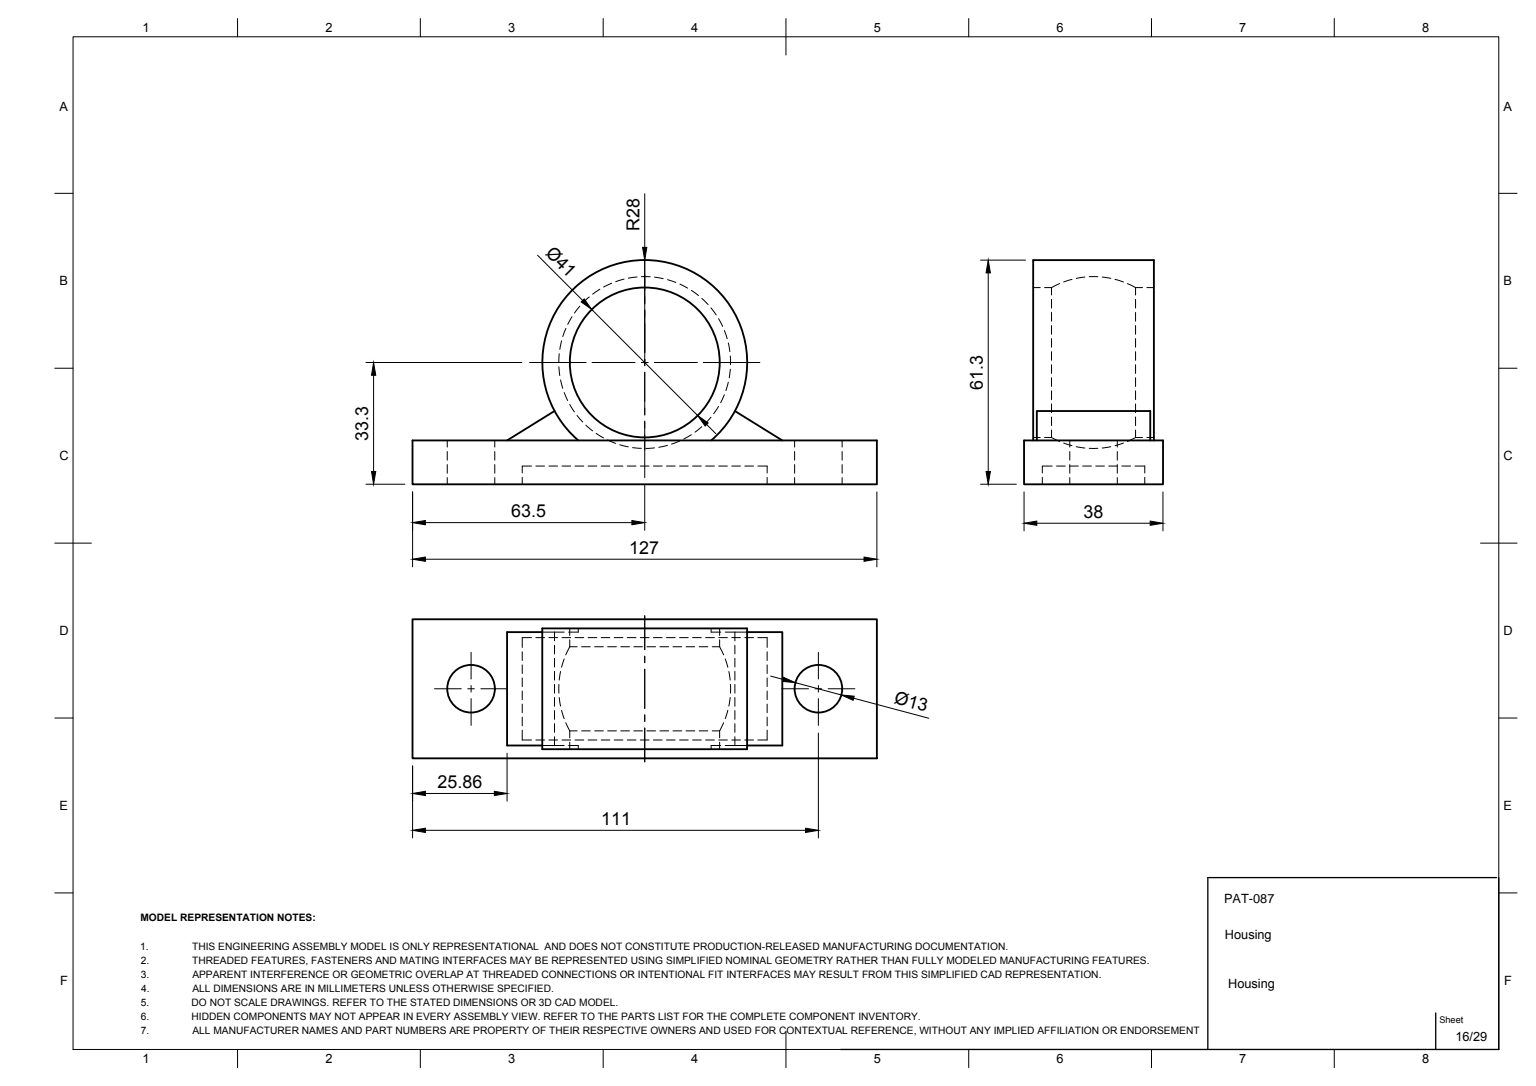
ISO-10303-21;
HEADER;
/* Generated by software containing ST-Developer
 * from STEP Tools, Inc. (www.steptools.com) 
 */

FILE_DESCRIPTION(
/* description */ ('Rigid flange shaft coupling assembly'),
/* implementation_level */ '2;1');

FILE_NAME(
/* name */ 'Housing.step',
/* time_stamp */ '2026-10-27T10:47:16-07:00',
/* author */ (''),
/* organization */ (''),
/* preprocessor_version */ 'ST-DEVELOPER v20.2',
/* originating_system */ 'Autodesk Translation Framework v15.17.0.0',
/* authorisation */ '');

FILE_SCHEMA (('AUTOMOTIVE_DESIGN { 1 0 10303 214 3 1 1 }'));
ENDSEC;

DATA;
#10=MECHANICAL_DESIGN_GEOMETRIC_PRESENTATION_REPRESENTATION('',(#407),#9141);
#340=SPHERICAL_SURFACE('',#5210,2.35);
#351=SHAPE_REPRESENTATION_RELATIONSHIP('SRR','None',#9286,#379);
#379=ADVANCED_BREP_SHAPE_REPRESENTATION('',(#436),#9121);
#407=STYLED_ITEM('',(#9479),#436);
#436=MANIFOLD_SOLID_BREP('Body1',#4761);
#485=FACE_BOUND('',#1109,.T.);
#486=FACE_BOUND('',#1110,.T.);
#487=FACE_BOUND('',#1118,.T.);
#488=FACE_BOUND('',#1119,.T.);
#489=FACE_BOUND('',#1120,.T.);
#490=FACE_BOUND('',#1123,.T.);
#491=FACE_BOUND('',#1125,.T.);
#492=FACE_BOUND('',#1138,.T.);
#493=FACE_BOUND('',#1139,.T.);
#494=FACE_BOUND('',#1140,.T.);
#608=PLANE('',#5212);
#609=PLANE('',#5214);
#610=PLANE('',#5216);
#611=PLANE('',#5218);
#612=PLANE('',#5219);
#613=PLANE('',#5221);
#614=PLANE('',#5222);
#615=PLANE('',#5228);
#616=PLANE('',#5229);
#617=PLANE('',#5230);
#618=PLANE('',#5231);
#619=PLANE('',#5232);
#620=PLANE('',#5233);
#621=PLANE('',#5234);
#622=PLANE('',#5239);
#623=PLANE('',#5240);
#624=PLANE('',#5241);
#625=PLANE('',#5242);
#626=PLANE('',#5243);
#802=FACE_OUTER_BOUND('',#1106,.T.);
#803=FACE_OUTER_BOUND('',#1107,.T.);
#804=FACE_OUTER_BOUND('',#1108,.T.);
#805=FACE_OUTER_BOUND('',#1111,.T.);
#806=FACE_OUTER_BOUND('',#1112,.T.);
#807=FACE_OUTER_BOUND('',#1113,.T.);
#808=FACE_OUTER_BOUND('',#1114,.T.);
#809=FACE_OUTER_BOUND('',#1115,.T.);
#810=FACE_OUTER_BOUND('',#1116,.T.);
#811=FACE_OUTER_BOUND('',#1117,.T.);
#812=FACE_OUTER_BOUND('',#1121,.T.);
#813=FACE_OUTER_BOUND('',#1122,.T.);
#814=FACE_OUTER_BOUND('',#1124,.T.);
#815=FACE_OUTER_BOUND('',#1126,.T.);
#816=FACE_OUTER_BOUND('',#1127,.T.);
#817=FACE_OUTER_BOUND('',#1128,.T.);
#818=FACE_OUTER_BOUND('',#1129,.T.);
#819=FACE_OUTER_BOUND('',#1130,.T.);
#820=FACE_OUTER_BOUND('',#1131,.T.);
#821=FACE_OUTER_BOUND('',#1132,.T.);
#822=FACE_OUTER_BOUND('',#1133,.T.);
#823=FACE_OUTER_BOUND('',#1134,.T.);
#824=FACE_OUTER_BOUND('',#1135,.T.);
#825=FACE_OUTER_BOUND('',#1136,.T.);
#826=FACE_OUTER_BOUND('',#1137,.T.);
#1106=EDGE_LOOP('',(#3483,#3484,#3485,#3486));
#1107=EDGE_LOOP('',(#3487,#3488,#3489,#3490));
#1108=EDGE_LOOP('',(#3491,#3492));
#1109=EDGE_LOOP('',(#3493));
#1110=EDGE_LOOP('',(#3494));
#1111=EDGE_LOOP('',(#3495,#3496,#3497));
#1112=EDGE_LOOP('',(#3498,#3499,#3500));
#1113=EDGE_LOOP('',(#3501,#3502,#3503));
#1114=EDGE_LOOP('',(#3504,#3505,#3506,#3507));
#1115=EDGE_LOOP('',(#3508,#3509,#3510));
#1116=EDGE_LOOP('',(#3511,#3512,#3513,#3514));
#1117=EDGE_LOOP('',(#3515,#3516,#3517,#3518));
#1118=EDGE_LOOP('',(#3519));
#1119=EDGE_LOOP('',(#3520));
#1120=EDGE_LOOP('',(#3521,#3522,#3523,#3524,#3525,#3526,#3527,#3528,#3529,
#3530,#3531,#3532));
#1121=EDGE_LOOP('',(#3533,#3534,#3535,#3536,#3537,#3538,#3539,#3540,#3541,
#3542,#3543,#3544));
#1122=EDGE_LOOP('',(#3545,#3546));
#1123=EDGE_LOOP('',(#3547));
#1124=EDGE_LOOP('',(#3548,#3549));
#1125=EDGE_LOOP('',(#3550));
#1126=EDGE_LOOP('',(#3551,#3552,#3553,#3554));
#1127=EDGE_LOOP('',(#3555,#3556,#3557,#3558));
#1128=EDGE_LOOP('',(#3559,#3560,#3561,#3562));
#1129=EDGE_LOOP('',(#3563,#3564,#3565,#3566));
#1130=EDGE_LOOP('',(#3567,#3568,#3569,#3570));
#1131=EDGE_LOOP('',(#3571,#3572,#3573,#3574));
#1132=EDGE_LOOP('',(#3575,#3576,#3577,#3578));
#1133=EDGE_LOOP('',(#3579,#3580,#3581,#3582));
#1134=EDGE_LOOP('',(#3583,#3584,#3585,#3586));
#1135=EDGE_LOOP('',(#3587,#3588,#3589,#3590));
#1136=EDGE_LOOP('',(#3591,#3592,#3593,#3594));
#1137=EDGE_LOOP('',(#3595,#3596,#3597,#3598));
#1138=EDGE_LOOP('',(#3599,#3600,#3601,#3602));
#1139=EDGE_LOOP('',(#3603));
#1140=EDGE_LOOP('',(#3604));
#1485=LINE('',#7360,#1830);
#1486=LINE('',#7366,#1831);
#1487=LINE('',#7375,#1832);
#1488=LINE('',#7377,#1833);
#1489=LINE('',#7382,#1834);
#1490=LINE('',#7385,#1835);
#1491=LINE('',#7389,#1836);
#1492=LINE('',#7392,#1837);
#1493=LINE('',#7394,#1838);
#1494=LINE('',#7395,#1839);
#1495=LINE('',#7399,#1840);
#1496=LINE('',#7401,#1841);
#1497=LINE('',#7404,#1842);
#1498=LINE('',#7405,#1843);
#1499=LINE('',#7409,#1844);
#1500=LINE('',#7411,#1845);
#1501=LINE('',#7413,#1846);
#1502=LINE('',#7414,#1847);
#1503=LINE('',#7420,#1848);
#1504=LINE('',#7422,#1849);
#1505=LINE('',#7423,#1850);
#1506=LINE('',#7425,#1851);
#1507=LINE('',#7427,#1852);
#1508=LINE('',#7428,#1853);
#1509=LINE('',#7437,#1854);
#1510=LINE('',#7439,#1855);
#1511=LINE('',#7441,#1856);
#1512=LINE('',#7442,#1857);
#1513=LINE('',#7445,#1858);
#1514=LINE('',#7447,#1859);
#1515=LINE('',#7448,#1860);
#1516=LINE('',#7451,#1861);
#1517=LINE('',#7453,#1862);
#1518=LINE('',#7454,#1863);
#1519=LINE('',#7456,#1864);
#1520=LINE('',#7457,#1865);
#1521=LINE('',#7462,#1866);
#1522=LINE('',#7466,#1867);
#1523=LINE('',#7470,#1868);
#1524=LINE('',#7471,#1869);
#1525=LINE('',#7472,#1870);
#1526=LINE('',#7475,#1871);
#1527=LINE('',#7476,#1872);
#1528=LINE('',#7479,#1873);
#1529=LINE('',#7480,#1874);
#1530=LINE('',#7482,#1875);
#1830=VECTOR('',#5948,2.05);
#1831=VECTOR('',#5955,2.05);
#1832=VECTOR('',#5964,1.);
#1833=VECTOR('',#5965,1.);
#1834=VECTOR('',#5970,1.);
#1835=VECTOR('',#5973,1.);
#1836=VECTOR('',#5976,1.);
#1837=VECTOR('',#5979,1.);
#1838=VECTOR('',#5982,1.);
#1839=VECTOR('',#5983,1.);
#1840=VECTOR('',#5986,1.);
#1841=VECTOR('',#5987,1.);
#1842=VECTOR('',#5992,1.);
#1843=VECTOR('',#5993,1.);
#1844=VECTOR('',#5996,1.);
#1845=VECTOR('',#5997,1.);
#1846=VECTOR('',#5998,1.);
#1847=VECTOR('',#5999,1.);
#1848=VECTOR('',#6004,1.);
#1849=VECTOR('',#6005,1.);
#1850=VECTOR('',#6006,1.);
#1851=VECTOR('',#6007,1.);
#1852=VECTOR('',#6008,1.);
#1853=VECTOR('',#6009,1.);
#1854=VECTOR('',#6022,1.);
#1855=VECTOR('',#6023,1.);
#1856=VECTOR('',#6024,1.);
#1857=VECTOR('',#6025,1.);
#1858=VECTOR('',#6028,1.);
#1859=VECTOR('',#6029,1.);
#1860=VECTOR('',#6030,1.);
#1861=VECTOR('',#6033,1.);
#1862=VECTOR('',#6034,1.);
#1863=VECTOR('',#6035,1.);
#1864=VECTOR('',#6038,1.);
#1865=VECTOR('',#6039,1.);
#1866=VECTOR('',#6046,0.65);
#1867=VECTOR('',#6051,0.65);
#1868=VECTOR('',#6054,1.);
#1869=VECTOR('',#6055,1.);
#1870=VECTOR('',#6056,1.);
#1871=VECTOR('',#6059,1.);
#1872=VECTOR('',#6060,1.);
#1873=VECTOR('',#6063,1.);
#1874=VECTOR('',#6064,1.);
#1875=VECTOR('',#6067,1.);
#2135=CIRCLE('',#5205,2.05);
#2136=CIRCLE('',#5206,2.05);
#2137=CIRCLE('',#5208,2.05);
#2138=CIRCLE('',#5209,2.05);
#2139=CIRCLE('',#5211,2.35);
#2140=CIRCLE('',#5213,2.8);
#2141=CIRCLE('',#5215,2.8);
#2142=CIRCLE('',#5217,2.8);
#2143=CIRCLE('',#5220,2.8);
#2144=CIRCLE('',#5223,0.65);
#2145=CIRCLE('',#5224,0.65);
#2146=CIRCLE('',#5226,2.8);
#2147=CIRCLE('',#5227,2.8);
#2148=CIRCLE('',#5236,0.65);
#2149=CIRCLE('',#5238,0.65);
#2356=VERTEX_POINT('',#7357);
#2357=VERTEX_POINT('',#7359);
#2358=VERTEX_POINT('',#7363);
#2359=VERTEX_POINT('',#7365);
#2360=VERTEX_POINT('',#7369);
#2361=VERTEX_POINT('',#7370);
#2362=VERTEX_POINT('',#7373);
#2363=VERTEX_POINT('',#7374);
#2364=VERTEX_POINT('',#7376);
#2365=VERTEX_POINT('',#7380);
#2366=VERTEX_POINT('',#7381);
#2367=VERTEX_POINT('',#7383);
#2368=VERTEX_POINT('',#7387);
#2369=VERTEX_POINT('',#7388);
#2370=VERTEX_POINT('',#7390);
#2371=VERTEX_POINT('',#7397);
#2372=VERTEX_POINT('',#7398);
#2373=VERTEX_POINT('',#7400);
#2374=VERTEX_POINT('',#7407);
#2375=VERTEX_POINT('',#7408);
#2376=VERTEX_POINT('',#7410);
#2377=VERTEX_POINT('',#7412);
#2378=VERTEX_POINT('',#7415);
#2379=VERTEX_POINT('',#7417);
#2380=VERTEX_POINT('',#7419);
#2381=VERTEX_POINT('',#7421);
#2382=VERTEX_POINT('',#7424);
#2383=VERTEX_POINT('',#7426);
#2384=VERTEX_POINT('',#7435);
#2385=VERTEX_POINT('',#7436);
#2386=VERTEX_POINT('',#7438);
#2387=VERTEX_POINT('',#7440);
#2388=VERTEX_POINT('',#7444);
#2389=VERTEX_POINT('',#7446);
#2390=VERTEX_POINT('',#7450);
#2391=VERTEX_POINT('',#7452);
#2392=VERTEX_POINT('',#7460);
#2393=VERTEX_POINT('',#7464);
#2394=VERTEX_POINT('',#7468);
#2395=VERTEX_POINT('',#7469);
#2396=VERTEX_POINT('',#7474);
#2397=VERTEX_POINT('',#7478);
#2785=EDGE_CURVE('',#2356,#2356,#2135,.T.);
#2786=EDGE_CURVE('',#2356,#2357,#1485,.T.);
#2787=EDGE_CURVE('',#2357,#2357,#2136,.T.);
#2788=EDGE_CURVE('',#2358,#2358,#2137,.T.);
#2789=EDGE_CURVE('',#2358,#2359,#1486,.T.);
#2790=EDGE_CURVE('',#2359,#2359,#2138,.T.);
#2791=EDGE_CURVE('',#2360,#2361,#2139,.T.);
#2792=EDGE_CURVE('',#2362,#2363,#1487,.T.);
#2793=EDGE_CURVE('',#2362,#2364,#1488,.T.);
#2794=EDGE_CURVE('',#2363,#2364,#2140,.T.);
#2795=EDGE_CURVE('',#2365,#2366,#1489,.T.);
#2796=EDGE_CURVE('',#2367,#2365,#2141,.T.);
#2797=EDGE_CURVE('',#2367,#2366,#1490,.T.);
#2798=EDGE_CURVE('',#2368,#2369,#1491,.T.);
#2799=EDGE_CURVE('',#2370,#2368,#2142,.T.);
#2800=EDGE_CURVE('',#2370,#2369,#1492,.T.);
#2801=EDGE_CURVE('',#2369,#2362,#1493,.T.);
#2802=EDGE_CURVE('',#2364,#2370,#1494,.T.);
#2803=EDGE_CURVE('',#2371,#2372,#1495,.T.);
#2804=EDGE_CURVE('',#2371,#2373,#1496,.T.);
#2805=EDGE_CURVE('',#2372,#2373,#2143,.T.);
#2806=EDGE_CURVE('',#2366,#2371,#1497,.T.);
#2807=EDGE_CURVE('',#2373,#2367,#1498,.T.);
#2808=EDGE_CURVE('',#2374,#2375,#1499,.T.);
#2809=EDGE_CURVE('',#2375,#2376,#1500,.T.);
#2810=EDGE_CURVE('',#2376,#2377,#1501,.T.);
#2811=EDGE_CURVE('',#2377,#2374,#1502,.T.);
#2812=EDGE_CURVE('',#2378,#2378,#2144,.T.);
#2813=EDGE_CURVE('',#2379,#2379,#2145,.T.);
#2814=EDGE_CURVE('',#2372,#2380,#1503,.T.);
#2815=EDGE_CURVE('',#2380,#2381,#1504,.T.);
#2816=EDGE_CURVE('',#2381,#2368,#1505,.T.);
#2817=EDGE_CURVE('',#2363,#2382,#1506,.T.);
#2818=EDGE_CURVE('',#2382,#2383,#1507,.T.);
#2819=EDGE_CURVE('',#2383,#2365,#1508,.T.);
#2820=EDGE_CURVE('',#2382,#2383,#2146,.T.);
#2821=EDGE_CURVE('',#2380,#2381,#2147,.T.);
#2822=EDGE_CURVE('',#2384,#2385,#1509,.T.);
#2823=EDGE_CURVE('',#2384,#2386,#1510,.T.);
#2824=EDGE_CURVE('',#2386,#2387,#1511,.T.);
#2825=EDGE_CURVE('',#2385,#2387,#1512,.T.);
#2826=EDGE_CURVE('',#2388,#2384,#1513,.T.);
#2827=EDGE_CURVE('',#2388,#2389,#1514,.T.);
#2828=EDGE_CURVE('',#2389,#2386,#1515,.T.);
#2829=EDGE_CURVE('',#2390,#2388,#1516,.T.);
#2830=EDGE_CURVE('',#2390,#2391,#1517,.T.);
#2831=EDGE_CURVE('',#2391,#2389,#1518,.T.);
#2832=EDGE_CURVE('',#2385,#2390,#1519,.T.);
#2833=EDGE_CURVE('',#2387,#2391,#1520,.T.);
#2834=EDGE_CURVE('',#2392,#2392,#2148,.T.);
#2835=EDGE_CURVE('',#2392,#2379,#1521,.T.);
#2836=EDGE_CURVE('',#2393,#2393,#2149,.T.);
#2837=EDGE_CURVE('',#2393,#2378,#1522,.T.);
#2838=EDGE_CURVE('',#2394,#2395,#1523,.T.);
#2839=EDGE_CURVE('',#2395,#2374,#1524,.T.);
#2840=EDGE_CURVE('',#2394,#2377,#1525,.T.);
#2841=EDGE_CURVE('',#2396,#2394,#1526,.T.);
#2842=EDGE_CURVE('',#2396,#2376,#1527,.T.);
#2843=EDGE_CURVE('',#2397,#2396,#1528,.T.);
#2844=EDGE_CURVE('',#2397,#2375,#1529,.T.);
#2845=EDGE_CURVE('',#2395,#2397,#1530,.T.);
#3483=ORIENTED_EDGE('',*,*,#2785,.F.);
#3484=ORIENTED_EDGE('',*,*,#2786,.T.);
#3485=ORIENTED_EDGE('',*,*,#2787,.F.);
#3486=ORIENTED_EDGE('',*,*,#2786,.F.);
#3487=ORIENTED_EDGE('',*,*,#2788,.F.);
#3488=ORIENTED_EDGE('',*,*,#2789,.T.);
#3489=ORIENTED_EDGE('',*,*,#2790,.F.);
#3490=ORIENTED_EDGE('',*,*,#2789,.F.);
#3491=ORIENTED_EDGE('',*,*,#2791,.T.);
#3492=ORIENTED_EDGE('',*,*,#2791,.F.);
#3493=ORIENTED_EDGE('',*,*,#2788,.T.);
#3494=ORIENTED_EDGE('',*,*,#2787,.T.);
#3495=ORIENTED_EDGE('',*,*,#2792,.F.);
#3496=ORIENTED_EDGE('',*,*,#2793,.T.);
#3497=ORIENTED_EDGE('',*,*,#2794,.F.);
#3498=ORIENTED_EDGE('',*,*,#2795,.F.);
#3499=ORIENTED_EDGE('',*,*,#2796,.F.);
#3500=ORIENTED_EDGE('',*,*,#2797,.T.);
#3501=ORIENTED_EDGE('',*,*,#2798,.F.);
#3502=ORIENTED_EDGE('',*,*,#2799,.F.);
#3503=ORIENTED_EDGE('',*,*,#2800,.T.);
#3504=ORIENTED_EDGE('',*,*,#2801,.F.);
#3505=ORIENTED_EDGE('',*,*,#2800,.F.);
#3506=ORIENTED_EDGE('',*,*,#2802,.F.);
#3507=ORIENTED_EDGE('',*,*,#2793,.F.);
#3508=ORIENTED_EDGE('',*,*,#2803,.F.);
#3509=ORIENTED_EDGE('',*,*,#2804,.T.);
#3510=ORIENTED_EDGE('',*,*,#2805,.F.);
#3511=ORIENTED_EDGE('',*,*,#2806,.F.);
#3512=ORIENTED_EDGE('',*,*,#2797,.F.);
#3513=ORIENTED_EDGE('',*,*,#2807,.F.);
#3514=ORIENTED_EDGE('',*,*,#2804,.F.);
#3515=ORIENTED_EDGE('',*,*,#2808,.T.);
#3516=ORIENTED_EDGE('',*,*,#2809,.T.);
#3517=ORIENTED_EDGE('',*,*,#2810,.T.);
#3518=ORIENTED_EDGE('',*,*,#2811,.T.);
#3519=ORIENTED_EDGE('',*,*,#2812,.T.);
#3520=ORIENTED_EDGE('',*,*,#2813,.T.);
#3521=ORIENTED_EDGE('',*,*,#2795,.T.);
#3522=ORIENTED_EDGE('',*,*,#2806,.T.);
#3523=ORIENTED_EDGE('',*,*,#2803,.T.);
#3524=ORIENTED_EDGE('',*,*,#2814,.T.);
#3525=ORIENTED_EDGE('',*,*,#2815,.T.);
#3526=ORIENTED_EDGE('',*,*,#2816,.T.);
#3527=ORIENTED_EDGE('',*,*,#2798,.T.);
#3528=ORIENTED_EDGE('',*,*,#2801,.T.);
#3529=ORIENTED_EDGE('',*,*,#2792,.T.);
#3530=ORIENTED_EDGE('',*,*,#2817,.T.);
#3531=ORIENTED_EDGE('',*,*,#2818,.T.);
#3532=ORIENTED_EDGE('',*,*,#2819,.T.);
#3533=ORIENTED_EDGE('',*,*,#2796,.T.);
#3534=ORIENTED_EDGE('',*,*,#2819,.F.);
#3535=ORIENTED_EDGE('',*,*,#2820,.F.);
#3536=ORIENTED_EDGE('',*,*,#2817,.F.);
#3537=ORIENTED_EDGE('',*,*,#2794,.T.);
#3538=ORIENTED_EDGE('',*,*,#2802,.T.);
#3539=ORIENTED_EDGE('',*,*,#2799,.T.);
#3540=ORIENTED_EDGE('',*,*,#2816,.F.);
#3541=ORIENTED_EDGE('',*,*,#2821,.F.);
#3542=ORIENTED_EDGE('',*,*,#2814,.F.);
#3543=ORIENTED_EDGE('',*,*,#2805,.T.);
#3544=ORIENTED_EDGE('',*,*,#2807,.T.);
#3545=ORIENTED_EDGE('',*,*,#2815,.F.);
#3546=ORIENTED_EDGE('',*,*,#2821,.T.);
#3547=ORIENTED_EDGE('',*,*,#2785,.T.);
#3548=ORIENTED_EDGE('',*,*,#2818,.F.);
#3549=ORIENTED_EDGE('',*,*,#2820,.T.);
#3550=ORIENTED_EDGE('',*,*,#2790,.T.);
#3551=ORIENTED_EDGE('',*,*,#2822,.F.);
#3552=ORIENTED_EDGE('',*,*,#2823,.T.);
#3553=ORIENTED_EDGE('',*,*,#2824,.T.);
#3554=ORIENTED_EDGE('',*,*,#2825,.F.);
#3555=ORIENTED_EDGE('',*,*,#2826,.F.);
#3556=ORIENTED_EDGE('',*,*,#2827,.T.);
#3557=ORIENTED_EDGE('',*,*,#2828,.T.);
#3558=ORIENTED_EDGE('',*,*,#2823,.F.);
#3559=ORIENTED_EDGE('',*,*,#2829,.F.);
#3560=ORIENTED_EDGE('',*,*,#2830,.T.);
#3561=ORIENTED_EDGE('',*,*,#2831,.T.);
#3562=ORIENTED_EDGE('',*,*,#2827,.F.);
#3563=ORIENTED_EDGE('',*,*,#2832,.F.);
#3564=ORIENTED_EDGE('',*,*,#2825,.T.);
#3565=ORIENTED_EDGE('',*,*,#2833,.T.);
#3566=ORIENTED_EDGE('',*,*,#2830,.F.);
#3567=ORIENTED_EDGE('',*,*,#2833,.F.);
#3568=ORIENTED_EDGE('',*,*,#2824,.F.);
#3569=ORIENTED_EDGE('',*,*,#2828,.F.);
#3570=ORIENTED_EDGE('',*,*,#2831,.F.);
#3571=ORIENTED_EDGE('',*,*,#2834,.F.);
#3572=ORIENTED_EDGE('',*,*,#2835,.T.);
#3573=ORIENTED_EDGE('',*,*,#2813,.F.);
#3574=ORIENTED_EDGE('',*,*,#2835,.F.);
#3575=ORIENTED_EDGE('',*,*,#2836,.F.);
#3576=ORIENTED_EDGE('',*,*,#2837,.T.);
#3577=ORIENTED_EDGE('',*,*,#2812,.F.);
#3578=ORIENTED_EDGE('',*,*,#2837,.F.);
#3579=ORIENTED_EDGE('',*,*,#2838,.T.);
#3580=ORIENTED_EDGE('',*,*,#2839,.T.);
#3581=ORIENTED_EDGE('',*,*,#2811,.F.);
#3582=ORIENTED_EDGE('',*,*,#2840,.F.);
#3583=ORIENTED_EDGE('',*,*,#2841,.T.);
#3584=ORIENTED_EDGE('',*,*,#2840,.T.);
#3585=ORIENTED_EDGE('',*,*,#2810,.F.);
#3586=ORIENTED_EDGE('',*,*,#2842,.F.);
#3587=ORIENTED_EDGE('',*,*,#2843,.T.);
#3588=ORIENTED_EDGE('',*,*,#2842,.T.);
#3589=ORIENTED_EDGE('',*,*,#2809,.F.);
#3590=ORIENTED_EDGE('',*,*,#2844,.F.);
#3591=ORIENTED_EDGE('',*,*,#2845,.T.);
#3592=ORIENTED_EDGE('',*,*,#2844,.T.);
#3593=ORIENTED_EDGE('',*,*,#2808,.F.);
#3594=ORIENTED_EDGE('',*,*,#2839,.F.);
#3595=ORIENTED_EDGE('',*,*,#2845,.F.);
#3596=ORIENTED_EDGE('',*,*,#2838,.F.);
#3597=ORIENTED_EDGE('',*,*,#2841,.F.);
#3598=ORIENTED_EDGE('',*,*,#2843,.F.);
#3599=ORIENTED_EDGE('',*,*,#2822,.T.);
#3600=ORIENTED_EDGE('',*,*,#2832,.T.);
#3601=ORIENTED_EDGE('',*,*,#2829,.T.);
#3602=ORIENTED_EDGE('',*,*,#2826,.T.);
#3603=ORIENTED_EDGE('',*,*,#2834,.T.);
#3604=ORIENTED_EDGE('',*,*,#2836,.T.);
#4419=CYLINDRICAL_SURFACE('',#5204,2.05);
#4420=CYLINDRICAL_SURFACE('',#5207,2.05);
#4421=CYLINDRICAL_SURFACE('',#5225,2.8);
#4422=CYLINDRICAL_SURFACE('',#5235,0.65);
#4423=CYLINDRICAL_SURFACE('',#5237,0.65);
#4538=ADVANCED_FACE('',(#802),#4419,.F.);
#4539=ADVANCED_FACE('',(#803),#4420,.F.);
#4540=ADVANCED_FACE('',(#804,#485,#486),#340,.F.);
#4541=ADVANCED_FACE('',(#805),#608,.T.);
#4542=ADVANCED_FACE('',(#806),#609,.T.);
#4543=ADVANCED_FACE('',(#807),#610,.T.);
#4544=ADVANCED_FACE('',(#808),#611,.T.);
#4545=ADVANCED_FACE('',(#809),#612,.T.);
#4546=ADVANCED_FACE('',(#810),#613,.T.);
#4547=ADVANCED_FACE('',(#811,#487,#488,#489),#614,.T.);
#4548=ADVANCED_FACE('',(#812),#4421,.T.);
#4549=ADVANCED_FACE('',(#813,#490),#615,.F.);
#4550=ADVANCED_FACE('',(#814,#491),#616,.T.);
#4551=ADVANCED_FACE('',(#815),#617,.F.);
#4552=ADVANCED_FACE('',(#816),#618,.F.);
#4553=ADVANCED_FACE('',(#817),#619,.F.);
#4554=ADVANCED_FACE('',(#818),#620,.F.);
#4555=ADVANCED_FACE('',(#819),#621,.F.);
#4556=ADVANCED_FACE('',(#820),#4422,.F.);
#4557=ADVANCED_FACE('',(#821),#4423,.F.);
#4558=ADVANCED_FACE('',(#822),#622,.T.);
#4559=ADVANCED_FACE('',(#823),#623,.T.);
#4560=ADVANCED_FACE('',(#824),#624,.T.);
#4561=ADVANCED_FACE('',(#825),#625,.T.);
#4562=ADVANCED_FACE('',(#826,#492,#493,#494),#626,.F.);
#4761=CLOSED_SHELL('',(#4538,#4539,#4540,#4541,#4542,#4543,#4544,#4545,
#4546,#4547,#4548,#4549,#4550,#4551,#4552,#4553,#4554,#4555,#4556,#4557,
#4558,#4559,#4560,#4561,#4562));
#5203=AXIS2_PLACEMENT_3D('',#7355,#5942,#5943);
#5204=AXIS2_PLACEMENT_3D('',#7356,#5944,#5945);
#5205=AXIS2_PLACEMENT_3D('',#7358,#5946,#5947);
#5206=AXIS2_PLACEMENT_3D('',#7361,#5949,#5950);
#5207=AXIS2_PLACEMENT_3D('',#7362,#5951,#5952);
#5208=AXIS2_PLACEMENT_3D('',#7364,#5953,#5954);
#5209=AXIS2_PLACEMENT_3D('',#7367,#5956,#5957);
#5210=AXIS2_PLACEMENT_3D('',#7368,#5958,#5959);
#5211=AXIS2_PLACEMENT_3D('',#7371,#5960,#5961);
#5212=AXIS2_PLACEMENT_3D('',#7372,#5962,#5963);
#5213=AXIS2_PLACEMENT_3D('',#7378,#5966,#5967);
#5214=AXIS2_PLACEMENT_3D('',#7379,#5968,#5969);
#5215=AXIS2_PLACEMENT_3D('',#7384,#5971,#5972);
#5216=AXIS2_PLACEMENT_3D('',#7386,#5974,#5975);
#5217=AXIS2_PLACEMENT_3D('',#7391,#5977,#5978);
#5218=AXIS2_PLACEMENT_3D('',#7393,#5980,#5981);
#5219=AXIS2_PLACEMENT_3D('',#7396,#5984,#5985);
#5220=AXIS2_PLACEMENT_3D('',#7402,#5988,#5989);
#5221=AXIS2_PLACEMENT_3D('',#7403,#5990,#5991);
#5222=AXIS2_PLACEMENT_3D('',#7406,#5994,#5995);
#5223=AXIS2_PLACEMENT_3D('',#7416,#6000,#6001);
#5224=AXIS2_PLACEMENT_3D('',#7418,#6002,#6003);
#5225=AXIS2_PLACEMENT_3D('',#7429,#6010,#6011);
#5226=AXIS2_PLACEMENT_3D('',#7430,#6012,#6013);
#5227=AXIS2_PLACEMENT_3D('',#7431,#6014,#6015);
#5228=AXIS2_PLACEMENT_3D('',#7432,#6016,#6017);
#5229=AXIS2_PLACEMENT_3D('',#7433,#6018,#6019);
#5230=AXIS2_PLACEMENT_3D('',#7434,#6020,#6021);
#5231=AXIS2_PLACEMENT_3D('',#7443,#6026,#6027);
#5232=AXIS2_PLACEMENT_3D('',#7449,#6031,#6032);
#5233=AXIS2_PLACEMENT_3D('',#7455,#6036,#6037);
#5234=AXIS2_PLACEMENT_3D('',#7458,#6040,#6041);
#5235=AXIS2_PLACEMENT_3D('',#7459,#6042,#6043);
#5236=AXIS2_PLACEMENT_3D('',#7461,#6044,#6045);
#5237=AXIS2_PLACEMENT_3D('',#7463,#6047,#6048);
#5238=AXIS2_PLACEMENT_3D('',#7465,#6049,#6050);
#5239=AXIS2_PLACEMENT_3D('',#7467,#6052,#6053);
#5240=AXIS2_PLACEMENT_3D('',#7473,#6057,#6058);
#5241=AXIS2_PLACEMENT_3D('',#7477,#6061,#6062);
#5242=AXIS2_PLACEMENT_3D('',#7481,#6065,#6066);
#5243=AXIS2_PLACEMENT_3D('',#7483,#6068,#6069);
#5942=DIRECTION('axis',(0.,0.,1.));
#5943=DIRECTION('refdir',(1.,0.,0.));
#5944=DIRECTION('center_axis',(0.,1.,0.));
#5945=DIRECTION('ref_axis',(1.,0.,0.));
#5946=DIRECTION('center_axis',(0.,1.,0.));
#5947=DIRECTION('ref_axis',(1.,0.,0.));
#5948=DIRECTION('',(0.,1.,0.));
#5949=DIRECTION('center_axis',(0.,-1.,0.));
#5950=DIRECTION('ref_axis',(1.,0.,0.));
#5951=DIRECTION('center_axis',(0.,1.,0.));
#5952=DIRECTION('ref_axis',(1.,0.,0.));
#5953=DIRECTION('center_axis',(0.,1.,0.));
#5954=DIRECTION('ref_axis',(1.,0.,0.));
#5955=DIRECTION('',(0.,1.,0.));
#5956=DIRECTION('center_axis',(0.,-1.,0.));
#5957=DIRECTION('ref_axis',(1.,0.,0.));
#5958=DIRECTION('center_axis',(6.12323399573677E-17,0.,1.));
#5959=DIRECTION('ref_axis',(1.,0.,0.));
#5960=DIRECTION('center_axis',(-1.22464679914735E-16,1.,0.));
#5961=DIRECTION('ref_axis',(-1.,-1.22464679914735E-16,0.));
#5962=DIRECTION('center_axis',(0.,1.,0.));
#5963=DIRECTION('ref_axis',(0.,0.,1.));
#5964=DIRECTION('',(1.,0.,0.));
#5965=DIRECTION('',(0.850265146687862,0.,0.526354614616295));
#5966=DIRECTION('center_axis',(0.,1.,0.));
#5967=DIRECTION('ref_axis',(1.,0.,0.));
#5968=DIRECTION('center_axis',(0.,1.,0.));
#5969=DIRECTION('ref_axis',(0.,0.,1.));
#5970=DIRECTION('',(1.,0.,0.));
#5971=DIRECTION('center_axis',(0.,1.,0.));
#5972=DIRECTION('ref_axis',(1.,0.,0.));
#5973=DIRECTION('',(0.850265146687862,0.,-0.526354614616295));
#5974=DIRECTION('center_axis',(0.,-1.,0.));
#5975=DIRECTION('ref_axis',(0.,0.,-1.));
#5976=DIRECTION('',(-1.,0.,0.));
#5977=DIRECTION('center_axis',(0.,-1.,0.));
#5978=DIRECTION('ref_axis',(1.,0.,0.));
#5979=DIRECTION('',(-0.850265146687862,0.,-0.526354614616295));
#5980=DIRECTION('center_axis',(-0.526354614616295,0.,0.850265146687862));
#5981=DIRECTION('ref_axis',(0.850265146687862,0.,0.526354614616295));
#5982=DIRECTION('',(0.,1.,0.));
#5983=DIRECTION('',(0.,-1.,0.));
#5984=DIRECTION('center_axis',(0.,-1.,0.));
#5985=DIRECTION('ref_axis',(0.,0.,-1.));
#5986=DIRECTION('',(-1.,0.,0.));
#5987=DIRECTION('',(-0.850265146687862,0.,0.526354614616295));
#5988=DIRECTION('center_axis',(0.,-1.,0.));
#5989=DIRECTION('ref_axis',(1.,0.,0.));
#5990=DIRECTION('center_axis',(0.526354614616295,0.,0.850265146687862));
#5991=DIRECTION('ref_axis',(0.850265146687862,0.,-0.526354614616295));
#5992=DIRECTION('',(0.,-1.,0.));
#5993=DIRECTION('',(0.,1.,0.));
#5994=DIRECTION('center_axis',(0.,0.,1.));
#5995=DIRECTION('ref_axis',(1.,0.,0.));
#5996=DIRECTION('',(0.,-1.,0.));
#5997=DIRECTION('',(1.,0.,0.));
#5998=DIRECTION('',(0.,1.,0.));
#5999=DIRECTION('',(-1.,0.,0.));
#6000=DIRECTION('center_axis',(0.,0.,-1.));
#6001=DIRECTION('ref_axis',(1.,0.,0.));
#6002=DIRECTION('center_axis',(0.,0.,-1.));
#6003=DIRECTION('ref_axis',(1.,0.,0.));
#6004=DIRECTION('',(0.,-1.,0.));
#6005=DIRECTION('',(-1.,0.,0.));
#6006=DIRECTION('',(0.,1.,0.));
#6007=DIRECTION('',(0.,1.,0.));
#6008=DIRECTION('',(1.,0.,0.));
#6009=DIRECTION('',(0.,-1.,0.));
#6010=DIRECTION('center_axis',(0.,1.,0.));
#6011=DIRECTION('ref_axis',(6.12323399573677E-17,0.,1.));
#6012=DIRECTION('center_axis',(0.,1.,0.));
#6013=DIRECTION('ref_axis',(1.,0.,0.));
#6014=DIRECTION('center_axis',(0.,-1.,0.));
#6015=DIRECTION('ref_axis',(1.,0.,0.));
#6016=DIRECTION('center_axis',(0.,1.,0.));
#6017=DIRECTION('ref_axis',(1.,0.,0.));
#6018=DIRECTION('center_axis',(0.,1.,0.));
#6019=DIRECTION('ref_axis',(1.,0.,0.));
#6020=DIRECTION('center_axis',(0.,1.,0.));
#6021=DIRECTION('ref_axis',(-1.,0.,0.));
#6022=DIRECTION('',(-1.,0.,0.));
#6023=DIRECTION('',(0.,0.,1.));
#6024=DIRECTION('',(-1.,0.,0.));
#6025=DIRECTION('',(0.,0.,1.));
#6026=DIRECTION('center_axis',(1.,0.,0.));
#6027=DIRECTION('ref_axis',(0.,1.,0.));
#6028=DIRECTION('',(0.,1.,0.));
#6029=DIRECTION('',(0.,0.,1.));
#6030=DIRECTION('',(0.,1.,0.));
#6031=DIRECTION('center_axis',(0.,-1.,0.));
#6032=DIRECTION('ref_axis',(1.,0.,0.));
#6033=DIRECTION('',(1.,0.,0.));
#6034=DIRECTION('',(0.,0.,1.));
#6035=DIRECTION('',(1.,0.,0.));
#6036=DIRECTION('center_axis',(-1.,0.,0.));
#6037=DIRECTION('ref_axis',(0.,-1.,0.));
#6038=DIRECTION('',(0.,-1.,0.));
#6039=DIRECTION('',(0.,-1.,0.));
#6040=DIRECTION('center_axis',(0.,0.,1.));
#6041=DIRECTION('ref_axis',(1.,0.,0.));
#6042=DIRECTION('center_axis',(0.,0.,1.));
#6043=DIRECTION('ref_axis',(1.,0.,0.));
#6044=DIRECTION('center_axis',(0.,0.,1.));
#6045=DIRECTION('ref_axis',(1.,0.,0.));
#6046=DIRECTION('',(0.,0.,1.));
#6047=DIRECTION('center_axis',(0.,0.,1.));
#6048=DIRECTION('ref_axis',(1.,0.,0.));
#6049=DIRECTION('center_axis',(0.,0.,1.));
#6050=DIRECTION('ref_axis',(1.,0.,0.));
#6051=DIRECTION('',(0.,0.,1.));
#6052=DIRECTION('center_axis',(0.,1.,0.));
#6053=DIRECTION('ref_axis',(-1.,0.,0.));
#6054=DIRECTION('',(-1.,0.,0.));
#6055=DIRECTION('',(0.,0.,1.));
#6056=DIRECTION('',(0.,0.,1.));
#6057=DIRECTION('center_axis',(1.,0.,0.));
#6058=DIRECTION('ref_axis',(0.,1.,0.));
#6059=DIRECTION('',(0.,1.,0.));
#6060=DIRECTION('',(0.,0.,1.));
#6061=DIRECTION('center_axis',(0.,-1.,0.));
#6062=DIRECTION('ref_axis',(1.,0.,0.));
#6063=DIRECTION('',(1.,0.,0.));
#6064=DIRECTION('',(0.,0.,1.));
#6065=DIRECTION('center_axis',(-1.,0.,0.));
#6066=DIRECTION('ref_axis',(0.,-1.,0.));
#6067=DIRECTION('',(0.,-1.,0.));
#6068=DIRECTION('center_axis',(0.,0.,1.));
#6069=DIRECTION('ref_axis',(1.,0.,0.));
#7355=CARTESIAN_POINT('',(0.,0.,0.));
#7356=CARTESIAN_POINT('Origin',(0.,0.,0.));
#7357=CARTESIAN_POINT('',(-2.05,-1.65,2.51052593825207E-16));
#7358=CARTESIAN_POINT('Origin',(0.,-1.65,0.));
#7359=CARTESIAN_POINT('',(-2.05,-1.14891252930761,-2.51052593825207E-16));
#7360=CARTESIAN_POINT('',(-2.05,0.,2.51052593825207E-16));
#7361=CARTESIAN_POINT('Origin',(0.,-1.14891252930761,0.));
#7362=CARTESIAN_POINT('Origin',(0.,0.,0.));
#7363=CARTESIAN_POINT('',(-2.05,1.14891252930761,2.51052593825207E-16));
#7364=CARTESIAN_POINT('Origin',(0.,1.14891252930761,0.));
#7365=CARTESIAN_POINT('',(-2.05,1.65,-2.51052593825207E-16));
#7366=CARTESIAN_POINT('',(-2.05,0.,2.51052593825207E-16));
#7367=CARTESIAN_POINT('Origin',(0.,1.65,0.));
#7368=CARTESIAN_POINT('Origin',(0.,0.,0.));
#7369=CARTESIAN_POINT('',(-1.43895998899814E-16,-1.76221774462768E-32,-2.35));
#7370=CARTESIAN_POINT('',(-1.43895998899814E-16,-1.76221774462768E-32,2.35));
#7371=CARTESIAN_POINT('Origin',(0.,0.,0.));
#7372=CARTESIAN_POINT('Origin',(0.,1.55,-1.49));
#7373=CARTESIAN_POINT('',(-3.76384615384615,1.55,-2.13));
#7374=CARTESIAN_POINT('',(-1.81744325908679,1.55,-2.13));
#7375=CARTESIAN_POINT('',(0.,1.55,-2.13));
#7376=CARTESIAN_POINT('',(-2.46585583768694,1.55,-1.32648218523477));
#7377=CARTESIAN_POINT('',(-1.68,1.55,-0.84));
#7378=CARTESIAN_POINT('Origin',(0.,1.55,0.));
#7379=CARTESIAN_POINT('Origin',(0.,1.55,-1.49));
#7380=CARTESIAN_POINT('',(1.81744325908679,1.55,-2.13));
#7381=CARTESIAN_POINT('',(3.76384615384615,1.55,-2.13));
#7382=CARTESIAN_POINT('',(0.,1.55,-2.13));
#7383=CARTESIAN_POINT('',(2.46585583768694,1.55,-1.32648218523477));
#7384=CARTESIAN_POINT('Origin',(0.,1.55,0.));
#7385=CARTESIAN_POINT('',(3.78,1.55,-2.14));
#7386=CARTESIAN_POINT('Origin',(0.,-1.55,-1.49));
#7387=CARTESIAN_POINT('',(-1.81744325908679,-1.55,-2.13));
#7388=CARTESIAN_POINT('',(-3.76384615384615,-1.55,-2.13));
#7389=CARTESIAN_POINT('',(0.,-1.55,-2.13));
#7390=CARTESIAN_POINT('',(-2.46585583768694,-1.55,-1.32648218523477));
#7391=CARTESIAN_POINT('Origin',(0.,-1.55,0.));
#7392=CARTESIAN_POINT('',(-1.68,-1.55,-0.84));
#7393=CARTESIAN_POINT('Origin',(-3.78,0.,-2.14));
#7394=CARTESIAN_POINT('',(-3.76384615384615,0.,-2.13));
#7395=CARTESIAN_POINT('',(-2.46585583768694,0.,-1.32648218523477));
#7396=CARTESIAN_POINT('Origin',(0.,-1.55,-1.49));
#7397=CARTESIAN_POINT('',(3.76384615384615,-1.55,-2.13));
#7398=CARTESIAN_POINT('',(1.81744325908679,-1.55,-2.13));
#7399=CARTESIAN_POINT('',(0.,-1.55,-2.13));
#7400=CARTESIAN_POINT('',(2.46585583768694,-1.55,-1.32648218523477));
#7401=CARTESIAN_POINT('',(3.78,-1.55,-2.14));
#7402=CARTESIAN_POINT('Origin',(0.,-1.55,0.));
#7403=CARTESIAN_POINT('Origin',(1.68,0.,-0.84));
#7404=CARTESIAN_POINT('',(3.76384615384615,0.,-2.13));
#7405=CARTESIAN_POINT('',(2.46585583768694,0.,-1.32648218523477));
#7406=CARTESIAN_POINT('Origin',(0.,0.,-2.13));
#7407=CARTESIAN_POINT('',(-6.35,1.9,-2.13));
#7408=CARTESIAN_POINT('',(-6.35,-1.9,-2.13));
#7409=CARTESIAN_POINT('',(-6.35,1.9,-2.13));
#7410=CARTESIAN_POINT('',(6.35,-1.9,-2.13));
#7411=CARTESIAN_POINT('',(-6.35,-1.9,-2.13));
#7412=CARTESIAN_POINT('',(6.35,1.9,-2.13));
#7413=CARTESIAN_POINT('',(6.35,-1.9,-2.13));
#7414=CARTESIAN_POINT('',(6.35,1.9,-2.13));
#7415=CARTESIAN_POINT('',(4.1,7.9602041944578E-17,-2.13));
#7416=CARTESIAN_POINT('Origin',(4.75,0.,-2.13));
#7417=CARTESIAN_POINT('',(-5.4,7.9602041944578E-17,-2.13));
#7418=CARTESIAN_POINT('Origin',(-4.75,0.,-2.13));
#7419=CARTESIAN_POINT('',(1.81744325908679,-1.65,-2.13));
#7420=CARTESIAN_POINT('',(1.81744325908679,0.,-2.13));
#7421=CARTESIAN_POINT('',(-1.81744325908679,-1.65,-2.13));
#7422=CARTESIAN_POINT('',(0.,-1.65,-2.13));
#7423=CARTESIAN_POINT('',(-1.81744325908679,0.,-2.13));
#7424=CARTESIAN_POINT('',(-1.81744325908679,1.65,-2.13));
#7425=CARTESIAN_POINT('',(-1.81744325908679,0.,-2.13));
#7426=CARTESIAN_POINT('',(1.81744325908679,1.65,-2.13));
#7427=CARTESIAN_POINT('',(0.,1.65,-2.13));
#7428=CARTESIAN_POINT('',(1.81744325908679,0.,-2.13));
#7429=CARTESIAN_POINT('Origin',(0.,0.,0.));
#7430=CARTESIAN_POINT('Origin',(0.,1.65,0.));
#7431=CARTESIAN_POINT('Origin',(0.,-1.65,0.));
#7432=CARTESIAN_POINT('Origin',(0.,-1.65,0.));
#7433=CARTESIAN_POINT('Origin',(0.,1.65,0.));
#7434=CARTESIAN_POINT('Origin',(3.35,1.4,-3.33));
#7435=CARTESIAN_POINT('',(3.35,1.4,-3.33));
#7436=CARTESIAN_POINT('',(-3.35,1.4,-3.33));
#7437=CARTESIAN_POINT('',(1.675,1.4,-3.33));
#7438=CARTESIAN_POINT('',(3.35,1.4,-2.83));
#7439=CARTESIAN_POINT('',(3.35,1.4,-3.33));
#7440=CARTESIAN_POINT('',(-3.35,1.4,-2.83));
#7441=CARTESIAN_POINT('',(3.35,1.4,-2.83));
#7442=CARTESIAN_POINT('',(-3.35,1.4,-3.33));
#7443=CARTESIAN_POINT('Origin',(3.35,-1.4,-3.33));
#7444=CARTESIAN_POINT('',(3.35,-1.4,-3.33));
#7445=CARTESIAN_POINT('',(3.35,-0.7,-3.33));
#7446=CARTESIAN_POINT('',(3.35,-1.4,-2.83));
#7447=CARTESIAN_POINT('',(3.35,-1.4,-3.33));
#7448=CARTESIAN_POINT('',(3.35,-1.4,-2.83));
#7449=CARTESIAN_POINT('Origin',(-3.35,-1.4,-3.33));
#7450=CARTESIAN_POINT('',(-3.35,-1.4,-3.33));
#7451=CARTESIAN_POINT('',(-1.675,-1.4,-3.33));
#7452=CARTESIAN_POINT('',(-3.35,-1.4,-2.83));
#7453=CARTESIAN_POINT('',(-3.35,-1.4,-3.33));
#7454=CARTESIAN_POINT('',(-3.35,-1.4,-2.83));
#7455=CARTESIAN_POINT('Origin',(-3.35,1.4,-3.33));
#7456=CARTESIAN_POINT('',(-3.35,0.7,-3.33));
#7457=CARTESIAN_POINT('',(-3.35,1.4,-2.83));
#7458=CARTESIAN_POINT('Origin',(0.,0.,-2.83));
#7459=CARTESIAN_POINT('Origin',(-4.75,0.,-3.33));
#7460=CARTESIAN_POINT('',(-5.4,-7.9602041944578E-17,-3.33));
#7461=CARTESIAN_POINT('Origin',(-4.75,0.,-3.33));
#7462=CARTESIAN_POINT('',(-5.4,-7.9602041944578E-17,-3.33));
#7463=CARTESIAN_POINT('Origin',(4.75,0.,-3.33));
#7464=CARTESIAN_POINT('',(4.1,-7.9602041944578E-17,-3.33));
#7465=CARTESIAN_POINT('Origin',(4.75,0.,-3.33));
#7466=CARTESIAN_POINT('',(4.1,-7.9602041944578E-17,-3.33));
#7467=CARTESIAN_POINT('Origin',(6.35,1.9,-3.33));
#7468=CARTESIAN_POINT('',(6.35,1.9,-3.33));
#7469=CARTESIAN_POINT('',(-6.35,1.9,-3.33));
#7470=CARTESIAN_POINT('',(6.35,1.9,-3.33));
#7471=CARTESIAN_POINT('',(-6.35,1.9,-3.33));
#7472=CARTESIAN_POINT('',(6.35,1.9,-3.33));
#7473=CARTESIAN_POINT('Origin',(6.35,-1.9,-3.33));
#7474=CARTESIAN_POINT('',(6.35,-1.9,-3.33));
#7475=CARTESIAN_POINT('',(6.35,-1.9,-3.33));
#7476=CARTESIAN_POINT('',(6.35,-1.9,-3.33));
#7477=CARTESIAN_POINT('Origin',(-6.35,-1.9,-3.33));
#7478=CARTESIAN_POINT('',(-6.35,-1.9,-3.33));
#7479=CARTESIAN_POINT('',(-6.35,-1.9,-3.33));
#7480=CARTESIAN_POINT('',(-6.35,-1.9,-3.33));
#7481=CARTESIAN_POINT('Origin',(-6.35,1.9,-3.33));
#7482=CARTESIAN_POINT('',(-6.35,1.9,-3.33));
#7483=CARTESIAN_POINT('Origin',(0.,0.,-3.33));
#9088=UNCERTAINTY_MEASURE_WITH_UNIT(LENGTH_MEASURE(0.001),#9142,
'DISTANCE_ACCURACY_VALUE',
'Maximum model space distance between geometric entities at asserted c
onnectivities');
#9108=UNCERTAINTY_MEASURE_WITH_UNIT(LENGTH_MEASURE(0.001),#9142,
'DISTANCE_ACCURACY_VALUE',
'Maximum model space distance between geometric entities at asserted c
onnectivities');
#9121=(
GEOMETRIC_REPRESENTATION_CONTEXT(3)
GLOBAL_UNCERTAINTY_ASSIGNED_CONTEXT((#9088))
GLOBAL_UNIT_ASSIGNED_CONTEXT((#9142,#9144,#9145))
REPRESENTATION_CONTEXT('','3D')
);
#9141=(
GEOMETRIC_REPRESENTATION_CONTEXT(3)
GLOBAL_UNCERTAINTY_ASSIGNED_CONTEXT((#9108))
GLOBAL_UNIT_ASSIGNED_CONTEXT((#9142,#9144,#9145))
REPRESENTATION_CONTEXT('','3D')
);
#9142=(
LENGTH_UNIT()
NAMED_UNIT(*)
SI_UNIT(.CENTI.,.METRE.)
);
#9144=(
NAMED_UNIT(*)
PLANE_ANGLE_UNIT()
SI_UNIT($,.RADIAN.)
);
#9145=(
NAMED_UNIT(*)
SI_UNIT($,.STERADIAN.)
SOLID_ANGLE_UNIT()
);
#9158=SHAPE_DEFINITION_REPRESENTATION(#9190,#9286);
#9190=PRODUCT_DEFINITION_SHAPE('',$,#9319);
#9286=SHAPE_REPRESENTATION('',(#5203),#9121);
#9306=PRODUCT_DEFINITION_CONTEXT('part definition',#9404,'design');
#9319=PRODUCT_DEFINITION('Housing','Housing',#9351,#9306);
#9351=PRODUCT_DEFINITION_FORMATION('',$,#9418);
#9404=APPLICATION_CONTEXT(
'Core Data for Automotive Mechanical Design Process');
#9405=PRODUCT_CONTEXT('part definition',#9404,'mechanical');
#9418=PRODUCT('Housing','Housing','Housing',(#9405));
#9473=COLOUR_RGB('Dark Blue',0.08,0.2,0.34);
#9474=FILL_AREA_STYLE_COLOUR('',#9473);
#9475=FILL_AREA_STYLE('',(#9474));
#9476=SURFACE_STYLE_FILL_AREA(#9475);
#9477=SURFACE_SIDE_STYLE('',(#9476));
#9478=SURFACE_STYLE_USAGE(.BOTH.,#9477);
#9479=PRESENTATION_STYLE_ASSIGNMENT((#9478));
ENDSEC;
END-ISO-10303-21;
